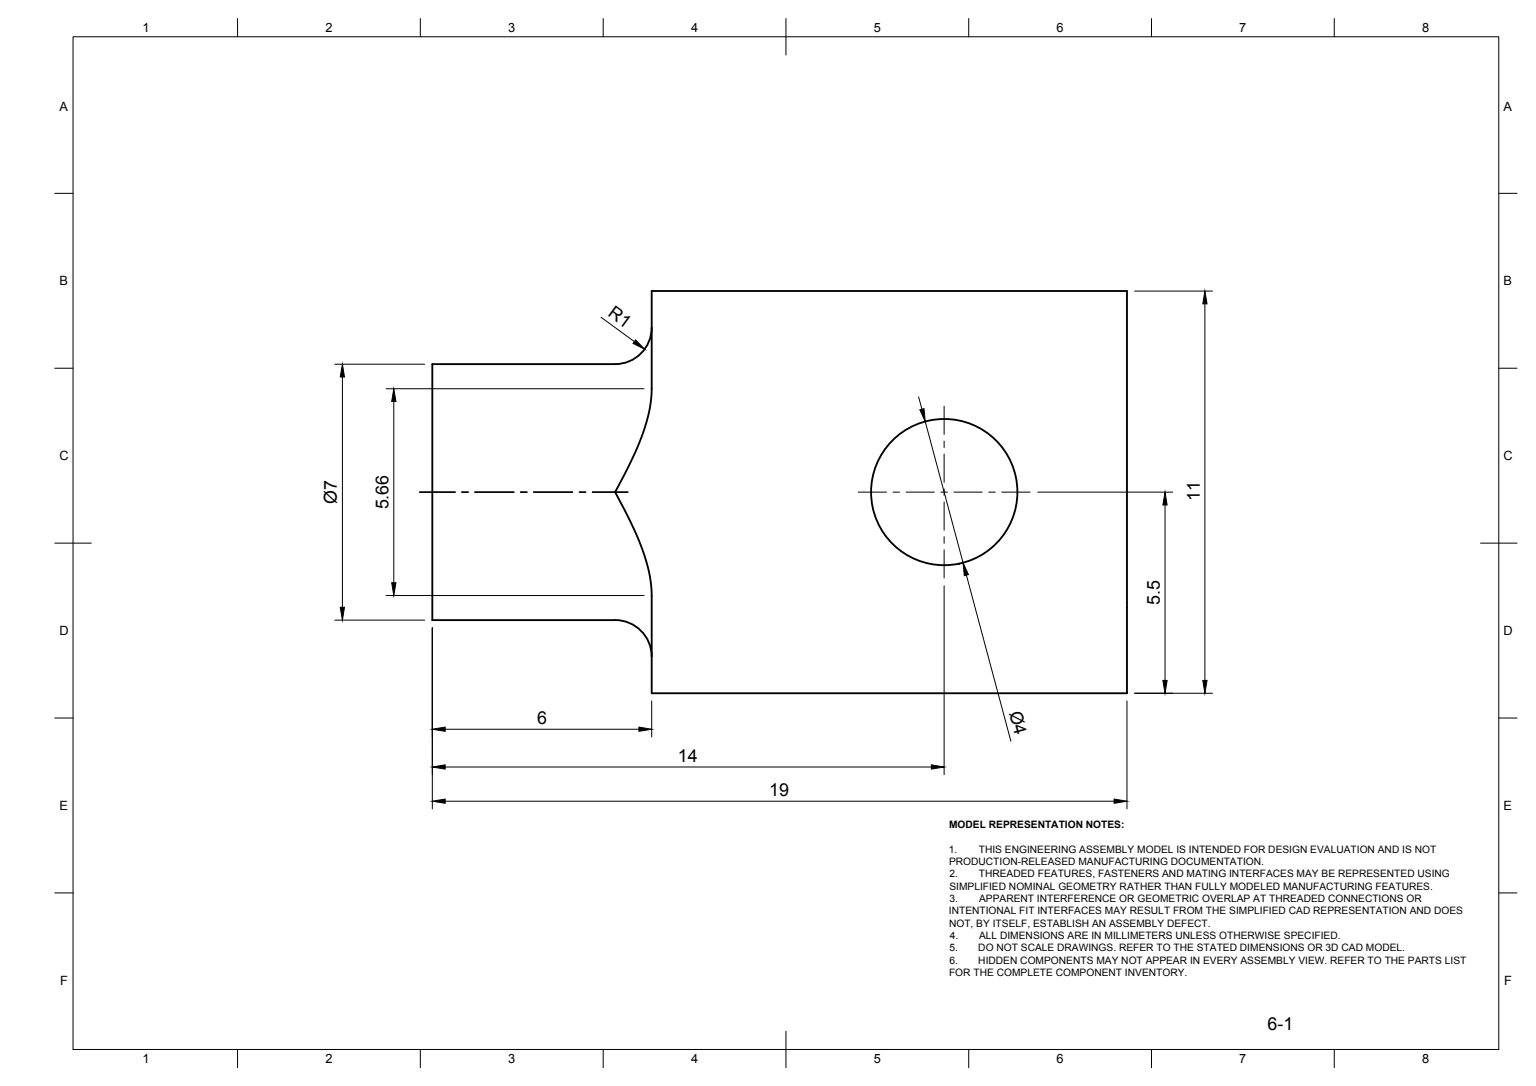
ISO-10303-21;
HEADER;
/* Generated by software containing ST-Developer
 * from STEP Tools, Inc. (www.steptools.com) 
 */

FILE_DESCRIPTION(
/* description */ (''),
/* implementation_level */ '2;1');

FILE_NAME(
/* name */ '6-1.step',
/* time_stamp */ '2026-10-06T01:16:10-07:00',
/* author */ (''),
/* organization */ (''),
/* preprocessor_version */ 'ST-DEVELOPER v20.2',
/* originating_system */ 'Autodesk Translation Framework v15.15.0.0',
/* authorisation */ '');

FILE_SCHEMA (('AUTOMOTIVE_DESIGN { 1 0 10303 214 3 1 1 }'));
ENDSEC;

DATA;
#10=MECHANICAL_DESIGN_GEOMETRIC_PRESENTATION_REPRESENTATION('',(#322,#323),#17113);
#144=TOROIDAL_SURFACE('',#6864,4.5,1.);
#145=TOROIDAL_SURFACE('',#6870,4.5,1.);
#217=B_SPLINE_CURVE_WITH_KNOTS('',3,(#16826,#16827,#16828,#16829),
 .UNSPECIFIED.,.F.,.F.,(4,4),(-0.288701302460675,0.),.UNSPECIFIED.);
#218=B_SPLINE_CURVE_WITH_KNOTS('',3,(#16830,#16831,#16832,#16833),
 .UNSPECIFIED.,.F.,.F.,(4,4),(-0.939904999188834,-0.651203696728158),
 .UNSPECIFIED.);
#219=B_SPLINE_CURVE_WITH_KNOTS('',3,(#16836,#16837,#16838,#16839),
 .UNSPECIFIED.,.F.,.F.,(4,4),(0.651203696728158,0.939904999188834),
 .UNSPECIFIED.);
#220=B_SPLINE_CURVE_WITH_KNOTS('',3,(#16849,#16850,#16851,#16852),
 .UNSPECIFIED.,.F.,.F.,(4,4),(0.,0.288701302460675),.UNSPECIFIED.);
#235=OPEN_SHELL('',(#5974,#5975));
#253=SHELL_BASED_SURFACE_MODEL('Body2',(#235));
#276=SHAPE_REPRESENTATION_RELATIONSHIP('SRR','None',#17202,#292);
#292=ADVANCED_BREP_SHAPE_REPRESENTATION('',(#342),#17109);
#322=STYLED_ITEM('',(#17298),#342);
#323=STYLED_ITEM('',(#17298),#253);
#342=MANIFOLD_SOLID_BREP('Body1',#6028);
#475=CYLINDRICAL_SURFACE('',#6844,2.);
#476=CYLINDRICAL_SURFACE('',#6857,1.75);
#477=CYLINDRICAL_SURFACE('',#6861,3.5);
#478=CYLINDRICAL_SURFACE('',#6867,2.);
#479=CYLINDRICAL_SURFACE('',#6871,2.);
#480=CYLINDRICAL_SURFACE('',#6872,5.5);
#481=CYLINDRICAL_SURFACE('',#6873,2.);
#482=CYLINDRICAL_SURFACE('',#6874,2.);
#483=CYLINDRICAL_SURFACE('',#6875,5.5);
#484=CYLINDRICAL_SURFACE('',#6876,2.);
#619=FACE_BOUND('',#1790,.T.);
#620=FACE_BOUND('',#1794,.T.);
#621=FACE_BOUND('',#1797,.T.);
#622=FACE_BOUND('',#1806,.T.);
#943=CIRCLE('',#6838,2.);
#944=CIRCLE('',#6839,5.5);
#945=CIRCLE('',#6840,2.);
#946=CIRCLE('',#6841,2.);
#947=CIRCLE('',#6842,5.5);
#948=CIRCLE('',#6843,2.);
#949=CIRCLE('',#6845,2.);
#950=CIRCLE('',#6847,1.75);
#951=CIRCLE('',#6849,4.5);
#952=CIRCLE('',#6850,2.);
#953=CIRCLE('',#6851,5.5);
#954=CIRCLE('',#6853,2.);
#955=CIRCLE('',#6854,4.5);
#956=CIRCLE('',#6855,2.);
#957=CIRCLE('',#6856,5.5);
#958=CIRCLE('',#6858,1.75);
#959=CIRCLE('',#6860,3.5);
#960=CIRCLE('',#6862,3.5);
#961=CIRCLE('',#6863,3.5);
#962=CIRCLE('',#6866,2.);
#963=CIRCLE('',#6868,2.);
#964=CIRCLE('',#6877,2.);
#965=CIRCLE('',#6878,2.);
#966=CIRCLE('',#6880,1.75);
#1308=FACE_OUTER_BOUND('',#1783,.T.);
#1309=FACE_OUTER_BOUND('',#1784,.T.);
#1310=FACE_OUTER_BOUND('',#1785,.T.);
#1311=FACE_OUTER_BOUND('',#1786,.T.);
#1312=FACE_OUTER_BOUND('',#1787,.T.);
#1313=FACE_OUTER_BOUND('',#1788,.T.);
#1314=FACE_OUTER_BOUND('',#1789,.T.);
#1315=FACE_OUTER_BOUND('',#1791,.T.);
#1316=FACE_OUTER_BOUND('',#1792,.T.);
#1317=FACE_OUTER_BOUND('',#1793,.T.);
#1318=FACE_OUTER_BOUND('',#1795,.T.);
#1319=FACE_OUTER_BOUND('',#1796,.T.);
#1320=FACE_OUTER_BOUND('',#1798,.T.);
#1321=FACE_OUTER_BOUND('',#1799,.T.);
#1322=FACE_OUTER_BOUND('',#1800,.T.);
#1323=FACE_OUTER_BOUND('',#1801,.T.);
#1324=FACE_OUTER_BOUND('',#1802,.T.);
#1325=FACE_OUTER_BOUND('',#1803,.T.);
#1326=FACE_OUTER_BOUND('',#1804,.T.);
#1327=FACE_OUTER_BOUND('',#1805,.T.);
#1783=EDGE_LOOP('',(#5252,#5253,#5254,#5255,#5256,#5257,#5258,#5259));
#1784=EDGE_LOOP('',(#5260,#5261,#5262,#5263));
#1785=EDGE_LOOP('',(#5264));
#1786=EDGE_LOOP('',(#5265,#5266,#5267,#5268,#5269,#5270));
#1787=EDGE_LOOP('',(#5271,#5272,#5273,#5274,#5275,#5276));
#1788=EDGE_LOOP('',(#5277,#5278,#5279,#5280));
#1789=EDGE_LOOP('',(#5281));
#1790=EDGE_LOOP('',(#5282));
#1791=EDGE_LOOP('',(#5283,#5284,#5285,#5286,#5287));
#1792=EDGE_LOOP('',(#5288,#5289,#5290,#5291));
#1793=EDGE_LOOP('',(#5292,#5293,#5294,#5295,#5296,#5297,#5298));
#1794=EDGE_LOOP('',(#5299));
#1795=EDGE_LOOP('',(#5300,#5301,#5302,#5303));
#1796=EDGE_LOOP('',(#5304,#5305,#5306,#5307,#5308,#5309,#5310));
#1797=EDGE_LOOP('',(#5311));
#1798=EDGE_LOOP('',(#5312,#5313,#5314,#5315));
#1799=EDGE_LOOP('',(#5316,#5317,#5318,#5319));
#1800=EDGE_LOOP('',(#5320,#5321,#5322,#5323));
#1801=EDGE_LOOP('',(#5324,#5325,#5326,#5327));
#1802=EDGE_LOOP('',(#5328,#5329,#5330,#5331));
#1803=EDGE_LOOP('',(#5332,#5333,#5334,#5335));
#1804=EDGE_LOOP('',(#5336,#5337,#5338,#5339));
#1805=EDGE_LOOP('',(#5340));
#1806=EDGE_LOOP('',(#5341));
#2160=LINE('',#16772,#2521);
#2161=LINE('',#16779,#2522);
#2162=LINE('',#16784,#2523);
#2163=LINE('',#16785,#2524);
#2164=LINE('',#16791,#2525);
#2165=LINE('',#16795,#2526);
#2166=LINE('',#16804,#2527);
#2167=LINE('',#16808,#2528);
#2168=LINE('',#16814,#2529);
#2169=LINE('',#16821,#2530);
#2170=LINE('',#16835,#2531);
#2171=LINE('',#16840,#2532);
#2172=LINE('',#16845,#2533);
#2173=LINE('',#16848,#2534);
#2174=LINE('',#16855,#2535);
#2175=LINE('',#16857,#2536);
#2176=LINE('',#16860,#2537);
#2177=LINE('',#16866,#2538);
#2521=VECTOR('',#8542,6.324555320337);
#2522=VECTOR('',#8549,6.324555320337);
#2523=VECTOR('',#8554,13.);
#2524=VECTOR('',#8555,13.);
#2525=VECTOR('',#8562,10.);
#2526=VECTOR('',#8565,10.);
#2527=VECTOR('',#8574,10.);
#2528=VECTOR('',#8577,10.);
#2529=VECTOR('',#8584,1.75);
#2530=VECTOR('',#8593,3.5);
#2531=VECTOR('',#8602,13.);
#2532=VECTOR('',#8603,13.);
#2533=VECTOR('',#8608,2.);
#2534=VECTOR('',#8613,13.);
#2535=VECTOR('',#8618,13.);
#2536=VECTOR('',#8621,13.);
#2537=VECTOR('',#8626,13.);
#2538=VECTOR('',#8633,2.);
#3017=VERTEX_POINT('',#16764);
#3018=VERTEX_POINT('',#16765);
#3019=VERTEX_POINT('',#16767);
#3020=VERTEX_POINT('',#16769);
#3021=VERTEX_POINT('',#16771);
#3022=VERTEX_POINT('',#16773);
#3023=VERTEX_POINT('',#16775);
#3024=VERTEX_POINT('',#16777);
#3025=VERTEX_POINT('',#16781);
#3026=VERTEX_POINT('',#16782);
#3027=VERTEX_POINT('',#16787);
#3028=VERTEX_POINT('',#16790);
#3029=VERTEX_POINT('',#16792);
#3030=VERTEX_POINT('',#16794);
#3031=VERTEX_POINT('',#16796);
#3032=VERTEX_POINT('',#16800);
#3033=VERTEX_POINT('',#16801);
#3034=VERTEX_POINT('',#16803);
#3035=VERTEX_POINT('',#16805);
#3036=VERTEX_POINT('',#16807);
#3037=VERTEX_POINT('',#16809);
#3038=VERTEX_POINT('',#16813);
#3039=VERTEX_POINT('',#16817);
#3040=VERTEX_POINT('',#16820);
#3041=VERTEX_POINT('',#16822);
#3042=VERTEX_POINT('',#16841);
#3043=VERTEX_POINT('',#16844);
#3044=VERTEX_POINT('',#16863);
#3045=VERTEX_POINT('',#16865);
#3046=VERTEX_POINT('',#16869);
#3786=EDGE_CURVE('',#3017,#3018,#943,.T.);
#3787=EDGE_CURVE('',#3018,#3019,#944,.T.);
#3788=EDGE_CURVE('',#3019,#3020,#945,.T.);
#3789=EDGE_CURVE('',#3020,#3021,#2160,.T.);
#3790=EDGE_CURVE('',#3021,#3022,#946,.T.);
#3791=EDGE_CURVE('',#3022,#3023,#947,.T.);
#3792=EDGE_CURVE('',#3023,#3024,#948,.T.);
#3793=EDGE_CURVE('',#3024,#3017,#2161,.T.);
#3794=EDGE_CURVE('',#3025,#3026,#949,.T.);
#3795=EDGE_CURVE('',#3018,#3025,#2162,.T.);
#3796=EDGE_CURVE('',#3017,#3026,#2163,.T.);
#3797=EDGE_CURVE('',#3027,#3027,#950,.T.);
#3798=EDGE_CURVE('',#3028,#3026,#2164,.T.);
#3799=EDGE_CURVE('',#3029,#3028,#951,.T.);
#3800=EDGE_CURVE('',#3030,#3029,#2165,.T.);
#3801=EDGE_CURVE('',#3030,#3031,#952,.T.);
#3802=EDGE_CURVE('',#3025,#3031,#953,.T.);
#3803=EDGE_CURVE('',#3032,#3033,#954,.T.);
#3804=EDGE_CURVE('',#3034,#3033,#2166,.T.);
#3805=EDGE_CURVE('',#3035,#3034,#955,.T.);
#3806=EDGE_CURVE('',#3036,#3035,#2167,.T.);
#3807=EDGE_CURVE('',#3036,#3037,#956,.T.);
#3808=EDGE_CURVE('',#3032,#3037,#957,.T.);
#3809=EDGE_CURVE('',#3027,#3038,#2168,.T.);
#3810=EDGE_CURVE('',#3038,#3038,#958,.T.);
#3811=EDGE_CURVE('',#3039,#3039,#959,.T.);
#3812=EDGE_CURVE('',#3039,#3040,#2169,.T.);
#3813=EDGE_CURVE('',#3040,#3041,#960,.T.);
#3814=EDGE_CURVE('',#3041,#3040,#961,.T.);
#3815=EDGE_CURVE('',#3028,#3040,#217,.T.);
#3816=EDGE_CURVE('',#3041,#3029,#218,.T.);
#3817=EDGE_CURVE('',#3020,#3030,#2170,.T.);
#3818=EDGE_CURVE('',#3034,#3041,#219,.T.);
#3819=EDGE_CURVE('',#3021,#3033,#2171,.T.);
#3820=EDGE_CURVE('',#3042,#3042,#962,.T.);
#3821=EDGE_CURVE('',#3042,#3043,#2172,.T.);
#3822=EDGE_CURVE('',#3043,#3043,#963,.T.);
#3823=EDGE_CURVE('',#3024,#3036,#2173,.T.);
#3824=EDGE_CURVE('',#3040,#3035,#220,.T.);
#3825=EDGE_CURVE('',#3023,#3037,#2174,.T.);
#3826=EDGE_CURVE('',#3022,#3032,#2175,.T.);
#3827=EDGE_CURVE('',#3019,#3031,#2176,.T.);
#3828=EDGE_CURVE('',#3044,#3044,#964,.T.);
#3829=EDGE_CURVE('',#3044,#3045,#2177,.T.);
#3830=EDGE_CURVE('',#3045,#3045,#965,.T.);
#3831=EDGE_CURVE('',#3046,#3046,#966,.T.);
#5252=ORIENTED_EDGE('',*,*,#3786,.T.);
#5253=ORIENTED_EDGE('',*,*,#3787,.T.);
#5254=ORIENTED_EDGE('',*,*,#3788,.T.);
#5255=ORIENTED_EDGE('',*,*,#3789,.T.);
#5256=ORIENTED_EDGE('',*,*,#3790,.T.);
#5257=ORIENTED_EDGE('',*,*,#3791,.T.);
#5258=ORIENTED_EDGE('',*,*,#3792,.T.);
#5259=ORIENTED_EDGE('',*,*,#3793,.T.);
#5260=ORIENTED_EDGE('',*,*,#3794,.F.);
#5261=ORIENTED_EDGE('',*,*,#3795,.F.);
#5262=ORIENTED_EDGE('',*,*,#3786,.F.);
#5263=ORIENTED_EDGE('',*,*,#3796,.T.);
#5264=ORIENTED_EDGE('',*,*,#3797,.T.);
#5265=ORIENTED_EDGE('',*,*,#3794,.T.);
#5266=ORIENTED_EDGE('',*,*,#3798,.F.);
#5267=ORIENTED_EDGE('',*,*,#3799,.F.);
#5268=ORIENTED_EDGE('',*,*,#3800,.F.);
#5269=ORIENTED_EDGE('',*,*,#3801,.T.);
#5270=ORIENTED_EDGE('',*,*,#3802,.F.);
#5271=ORIENTED_EDGE('',*,*,#3803,.T.);
#5272=ORIENTED_EDGE('',*,*,#3804,.F.);
#5273=ORIENTED_EDGE('',*,*,#3805,.F.);
#5274=ORIENTED_EDGE('',*,*,#3806,.F.);
#5275=ORIENTED_EDGE('',*,*,#3807,.T.);
#5276=ORIENTED_EDGE('',*,*,#3808,.F.);
#5277=ORIENTED_EDGE('',*,*,#3797,.F.);
#5278=ORIENTED_EDGE('',*,*,#3809,.T.);
#5279=ORIENTED_EDGE('',*,*,#3810,.F.);
#5280=ORIENTED_EDGE('',*,*,#3809,.F.);
#5281=ORIENTED_EDGE('',*,*,#3811,.T.);
#5282=ORIENTED_EDGE('',*,*,#3810,.T.);
#5283=ORIENTED_EDGE('',*,*,#3811,.F.);
#5284=ORIENTED_EDGE('',*,*,#3812,.T.);
#5285=ORIENTED_EDGE('',*,*,#3813,.T.);
#5286=ORIENTED_EDGE('',*,*,#3814,.T.);
#5287=ORIENTED_EDGE('',*,*,#3812,.F.);
#5288=ORIENTED_EDGE('',*,*,#3799,.T.);
#5289=ORIENTED_EDGE('',*,*,#3815,.T.);
#5290=ORIENTED_EDGE('',*,*,#3814,.F.);
#5291=ORIENTED_EDGE('',*,*,#3816,.T.);
#5292=ORIENTED_EDGE('',*,*,#3817,.T.);
#5293=ORIENTED_EDGE('',*,*,#3800,.T.);
#5294=ORIENTED_EDGE('',*,*,#3816,.F.);
#5295=ORIENTED_EDGE('',*,*,#3818,.F.);
#5296=ORIENTED_EDGE('',*,*,#3804,.T.);
#5297=ORIENTED_EDGE('',*,*,#3819,.F.);
#5298=ORIENTED_EDGE('',*,*,#3789,.F.);
#5299=ORIENTED_EDGE('',*,*,#3820,.T.);
#5300=ORIENTED_EDGE('',*,*,#3820,.F.);
#5301=ORIENTED_EDGE('',*,*,#3821,.T.);
#5302=ORIENTED_EDGE('',*,*,#3822,.T.);
#5303=ORIENTED_EDGE('',*,*,#3821,.F.);
#5304=ORIENTED_EDGE('',*,*,#3796,.F.);
#5305=ORIENTED_EDGE('',*,*,#3793,.F.);
#5306=ORIENTED_EDGE('',*,*,#3823,.T.);
#5307=ORIENTED_EDGE('',*,*,#3806,.T.);
#5308=ORIENTED_EDGE('',*,*,#3824,.F.);
#5309=ORIENTED_EDGE('',*,*,#3815,.F.);
#5310=ORIENTED_EDGE('',*,*,#3798,.T.);
#5311=ORIENTED_EDGE('',*,*,#3822,.F.);
#5312=ORIENTED_EDGE('',*,*,#3813,.F.);
#5313=ORIENTED_EDGE('',*,*,#3824,.T.);
#5314=ORIENTED_EDGE('',*,*,#3805,.T.);
#5315=ORIENTED_EDGE('',*,*,#3818,.T.);
#5316=ORIENTED_EDGE('',*,*,#3807,.F.);
#5317=ORIENTED_EDGE('',*,*,#3823,.F.);
#5318=ORIENTED_EDGE('',*,*,#3792,.F.);
#5319=ORIENTED_EDGE('',*,*,#3825,.T.);
#5320=ORIENTED_EDGE('',*,*,#3826,.T.);
#5321=ORIENTED_EDGE('',*,*,#3808,.T.);
#5322=ORIENTED_EDGE('',*,*,#3825,.F.);
#5323=ORIENTED_EDGE('',*,*,#3791,.F.);
#5324=ORIENTED_EDGE('',*,*,#3803,.F.);
#5325=ORIENTED_EDGE('',*,*,#3826,.F.);
#5326=ORIENTED_EDGE('',*,*,#3790,.F.);
#5327=ORIENTED_EDGE('',*,*,#3819,.T.);
#5328=ORIENTED_EDGE('',*,*,#3801,.F.);
#5329=ORIENTED_EDGE('',*,*,#3817,.F.);
#5330=ORIENTED_EDGE('',*,*,#3788,.F.);
#5331=ORIENTED_EDGE('',*,*,#3827,.T.);
#5332=ORIENTED_EDGE('',*,*,#3795,.T.);
#5333=ORIENTED_EDGE('',*,*,#3802,.T.);
#5334=ORIENTED_EDGE('',*,*,#3827,.F.);
#5335=ORIENTED_EDGE('',*,*,#3787,.F.);
#5336=ORIENTED_EDGE('',*,*,#3828,.F.);
#5337=ORIENTED_EDGE('',*,*,#3829,.T.);
#5338=ORIENTED_EDGE('',*,*,#3830,.T.);
#5339=ORIENTED_EDGE('',*,*,#3829,.F.);
#5340=ORIENTED_EDGE('',*,*,#3830,.F.);
#5341=ORIENTED_EDGE('',*,*,#3831,.F.);
#5627=PLANE('',#6837);
#5628=PLANE('',#6846);
#5629=PLANE('',#6848);
#5630=PLANE('',#6852);
#5631=PLANE('',#6859);
#5632=PLANE('',#6865);
#5633=PLANE('',#6869);
#5634=PLANE('',#6879);
#5956=ADVANCED_FACE('',(#1308),#5627,.T.);
#5957=ADVANCED_FACE('',(#1309),#475,.T.);
#5958=ADVANCED_FACE('',(#1310),#5628,.F.);
#5959=ADVANCED_FACE('',(#1311),#5629,.F.);
#5960=ADVANCED_FACE('',(#1312),#5630,.F.);
#5961=ADVANCED_FACE('',(#1313),#476,.F.);
#5962=ADVANCED_FACE('',(#1314,#619),#5631,.T.);
#5963=ADVANCED_FACE('',(#1315),#477,.T.);
#5964=ADVANCED_FACE('',(#1316),#144,.F.);
#5965=ADVANCED_FACE('',(#1317,#620),#5632,.T.);
#5966=ADVANCED_FACE('',(#1318),#478,.F.);
#5967=ADVANCED_FACE('',(#1319,#621),#5633,.T.);
#5968=ADVANCED_FACE('',(#1320),#145,.F.);
#5969=ADVANCED_FACE('',(#1321),#479,.T.);
#5970=ADVANCED_FACE('',(#1322),#480,.T.);
#5971=ADVANCED_FACE('',(#1323),#481,.T.);
#5972=ADVANCED_FACE('',(#1324),#482,.T.);
#5973=ADVANCED_FACE('',(#1325),#483,.T.);
#5974=ADVANCED_FACE('',(#1326),#484,.T.);
#5975=ADVANCED_FACE('',(#1327,#622),#5634,.F.);
#6028=CLOSED_SHELL('',(#5956,#5957,#5958,#5959,#5960,#5961,#5962,#5963,
#5964,#5965,#5966,#5967,#5968,#5969,#5970,#5971,#5972,#5973));
#6836=AXIS2_PLACEMENT_3D('',#16762,#8532,#8533);
#6837=AXIS2_PLACEMENT_3D('',#16763,#8534,#8535);
#6838=AXIS2_PLACEMENT_3D('',#16766,#8536,#8537);
#6839=AXIS2_PLACEMENT_3D('',#16768,#8538,#8539);
#6840=AXIS2_PLACEMENT_3D('',#16770,#8540,#8541);
#6841=AXIS2_PLACEMENT_3D('',#16774,#8543,#8544);
#6842=AXIS2_PLACEMENT_3D('',#16776,#8545,#8546);
#6843=AXIS2_PLACEMENT_3D('',#16778,#8547,#8548);
#6844=AXIS2_PLACEMENT_3D('',#16780,#8550,#8551);
#6845=AXIS2_PLACEMENT_3D('',#16783,#8552,#8553);
#6846=AXIS2_PLACEMENT_3D('',#16786,#8556,#8557);
#6847=AXIS2_PLACEMENT_3D('',#16788,#8558,#8559);
#6848=AXIS2_PLACEMENT_3D('',#16789,#8560,#8561);
#6849=AXIS2_PLACEMENT_3D('',#16793,#8563,#8564);
#6850=AXIS2_PLACEMENT_3D('',#16797,#8566,#8567);
#6851=AXIS2_PLACEMENT_3D('',#16798,#8568,#8569);
#6852=AXIS2_PLACEMENT_3D('',#16799,#8570,#8571);
#6853=AXIS2_PLACEMENT_3D('',#16802,#8572,#8573);
#6854=AXIS2_PLACEMENT_3D('',#16806,#8575,#8576);
#6855=AXIS2_PLACEMENT_3D('',#16810,#8578,#8579);
#6856=AXIS2_PLACEMENT_3D('',#16811,#8580,#8581);
#6857=AXIS2_PLACEMENT_3D('',#16812,#8582,#8583);
#6858=AXIS2_PLACEMENT_3D('',#16815,#8585,#8586);
#6859=AXIS2_PLACEMENT_3D('',#16816,#8587,#8588);
#6860=AXIS2_PLACEMENT_3D('',#16818,#8589,#8590);
#6861=AXIS2_PLACEMENT_3D('',#16819,#8591,#8592);
#6862=AXIS2_PLACEMENT_3D('',#16823,#8594,#8595);
#6863=AXIS2_PLACEMENT_3D('',#16824,#8596,#8597);
#6864=AXIS2_PLACEMENT_3D('',#16825,#8598,#8599);
#6865=AXIS2_PLACEMENT_3D('',#16834,#8600,#8601);
#6866=AXIS2_PLACEMENT_3D('',#16842,#8604,#8605);
#6867=AXIS2_PLACEMENT_3D('',#16843,#8606,#8607);
#6868=AXIS2_PLACEMENT_3D('',#16846,#8609,#8610);
#6869=AXIS2_PLACEMENT_3D('',#16847,#8611,#8612);
#6870=AXIS2_PLACEMENT_3D('',#16853,#8614,#8615);
#6871=AXIS2_PLACEMENT_3D('',#16854,#8616,#8617);
#6872=AXIS2_PLACEMENT_3D('',#16856,#8619,#8620);
#6873=AXIS2_PLACEMENT_3D('',#16858,#8622,#8623);
#6874=AXIS2_PLACEMENT_3D('',#16859,#8624,#8625);
#6875=AXIS2_PLACEMENT_3D('',#16861,#8627,#8628);
#6876=AXIS2_PLACEMENT_3D('',#16862,#8629,#8630);
#6877=AXIS2_PLACEMENT_3D('',#16864,#8631,#8632);
#6878=AXIS2_PLACEMENT_3D('',#16867,#8634,#8635);
#6879=AXIS2_PLACEMENT_3D('',#16868,#8636,#8637);
#6880=AXIS2_PLACEMENT_3D('',#16870,#8638,#8639);
#8532=DIRECTION('axis',(0.,0.,1.));
#8533=DIRECTION('refdir',(1.,0.,0.));
#8534=DIRECTION('center_axis',(0.,1.,0.));
#8535=DIRECTION('ref_axis',(1.,0.,0.));
#8536=DIRECTION('center_axis',(0.,1.,0.));
#8537=DIRECTION('ref_axis',(0.,0.,1.));
#8538=DIRECTION('center_axis',(0.,1.,0.));
#8539=DIRECTION('ref_axis',(0.903507902905271,0.,0.428571428571386));
#8540=DIRECTION('center_axis',(0.,1.,0.));
#8541=DIRECTION('ref_axis',(0.903507902905271,0.,-0.428571428571386));
#8542=DIRECTION('',(-1.,0.,0.));
#8543=DIRECTION('center_axis',(0.,1.,0.));
#8544=DIRECTION('ref_axis',(0.,0.,-1.));
#8545=DIRECTION('center_axis',(0.,1.,0.));
#8546=DIRECTION('ref_axis',(-0.903507902905271,0.,-0.428571428571386));
#8547=DIRECTION('center_axis',(0.,1.,0.));
#8548=DIRECTION('ref_axis',(-0.903507902905271,0.,0.428571428571386));
#8549=DIRECTION('',(1.,0.,0.));
#8550=DIRECTION('center_axis',(0.,-1.,0.));
#8551=DIRECTION('ref_axis',(0.903507902905271,0.,0.428571428571386));
#8552=DIRECTION('center_axis',(0.,-1.,0.));
#8553=DIRECTION('ref_axis',(0.903507902905271,0.,0.428571428571386));
#8554=DIRECTION('',(0.,-1.,0.));
#8555=DIRECTION('',(0.,-1.,0.));
#8556=DIRECTION('center_axis',(0.,1.,0.));
#8557=DIRECTION('ref_axis',(1.,0.,0.));
#8558=DIRECTION('center_axis',(0.,-1.,0.));
#8559=DIRECTION('ref_axis',(0.,0.,1.));
#8560=DIRECTION('center_axis',(0.,1.,0.));
#8561=DIRECTION('ref_axis',(1.,0.,0.));
#8562=DIRECTION('',(1.,0.,0.));
#8563=DIRECTION('center_axis',(0.,-1.,0.));
#8564=DIRECTION('ref_axis',(0.628539361054693,0.,-0.777777777777791));
#8565=DIRECTION('',(-1.,0.,0.));
#8566=DIRECTION('center_axis',(0.,-1.,0.));
#8567=DIRECTION('ref_axis',(0.,0.,-1.));
#8568=DIRECTION('center_axis',(0.,1.,0.));
#8569=DIRECTION('ref_axis',(0.903507902905271,0.,0.428571428571386));
#8570=DIRECTION('center_axis',(0.,1.,0.));
#8571=DIRECTION('ref_axis',(1.,0.,0.));
#8572=DIRECTION('center_axis',(0.,-1.,0.));
#8573=DIRECTION('ref_axis',(-0.903507902905271,0.,-0.428571428571386));
#8574=DIRECTION('',(-1.,0.,0.));
#8575=DIRECTION('center_axis',(0.,-1.,0.));
#8576=DIRECTION('ref_axis',(-0.628539361054693,0.,0.777777777777791));
#8577=DIRECTION('',(1.,0.,0.));
#8578=DIRECTION('center_axis',(0.,-1.,0.));
#8579=DIRECTION('ref_axis',(0.,0.,1.));
#8580=DIRECTION('center_axis',(0.,1.,0.));
#8581=DIRECTION('ref_axis',(-0.903507902905271,0.,-0.428571428571386));
#8582=DIRECTION('center_axis',(0.,-1.,0.));
#8583=DIRECTION('ref_axis',(0.,0.,-1.));
#8584=DIRECTION('',(0.,-1.,0.));
#8585=DIRECTION('center_axis',(0.,1.,0.));
#8586=DIRECTION('ref_axis',(0.,0.,-1.));
#8587=DIRECTION('center_axis',(0.,-1.,0.));
#8588=DIRECTION('ref_axis',(0.,0.,-1.));
#8589=DIRECTION('center_axis',(0.,-1.,0.));
#8590=DIRECTION('ref_axis',(0.,0.,-1.));
#8591=DIRECTION('center_axis',(0.,-1.,0.));
#8592=DIRECTION('ref_axis',(0.,0.,-1.));
#8593=DIRECTION('',(0.,1.,0.));
#8594=DIRECTION('center_axis',(0.,-1.,0.));
#8595=DIRECTION('ref_axis',(0.,0.,1.));
#8596=DIRECTION('center_axis',(0.,-1.,0.));
#8597=DIRECTION('ref_axis',(0.,0.,-1.));
#8598=DIRECTION('center_axis',(0.,-1.,0.));
#8599=DIRECTION('ref_axis',(1.,0.,-1.75640751942652E-17));
#8600=DIRECTION('center_axis',(0.,0.,-1.));
#8601=DIRECTION('ref_axis',(-1.,0.,0.));
#8602=DIRECTION('',(0.,-1.,0.));
#8603=DIRECTION('',(0.,-1.,0.));
#8604=DIRECTION('center_axis',(0.,0.,1.));
#8605=DIRECTION('ref_axis',(0.,-1.,0.));
#8606=DIRECTION('center_axis',(0.,0.,1.));
#8607=DIRECTION('ref_axis',(0.,-1.,0.));
#8608=DIRECTION('',(0.,0.,1.));
#8609=DIRECTION('center_axis',(0.,0.,1.));
#8610=DIRECTION('ref_axis',(0.,-1.,0.));
#8611=DIRECTION('center_axis',(0.,0.,1.));
#8612=DIRECTION('ref_axis',(1.,0.,0.));
#8613=DIRECTION('',(0.,-1.,0.));
#8614=DIRECTION('center_axis',(0.,-1.,0.));
#8615=DIRECTION('ref_axis',(-1.,0.,-2.27465615787459E-16));
#8616=DIRECTION('center_axis',(0.,-1.,0.));
#8617=DIRECTION('ref_axis',(0.,0.,1.));
#8618=DIRECTION('',(0.,-1.,0.));
#8619=DIRECTION('center_axis',(0.,1.,0.));
#8620=DIRECTION('ref_axis',(-1.,0.,-1.22464679914735E-16));
#8621=DIRECTION('',(0.,-1.,0.));
#8622=DIRECTION('center_axis',(0.,-1.,0.));
#8623=DIRECTION('ref_axis',(-0.903507902905271,0.,-0.428571428571386));
#8624=DIRECTION('center_axis',(0.,-1.,0.));
#8625=DIRECTION('ref_axis',(0.,0.,-1.));
#8626=DIRECTION('',(0.,-1.,0.));
#8627=DIRECTION('center_axis',(0.,1.,0.));
#8628=DIRECTION('ref_axis',(1.,0.,0.));
#8629=DIRECTION('center_axis',(0.,-1.,0.));
#8630=DIRECTION('ref_axis',(1.,0.,0.));
#8631=DIRECTION('center_axis',(0.,-1.,0.));
#8632=DIRECTION('ref_axis',(-1.,0.,0.));
#8633=DIRECTION('',(0.,1.,0.));
#8634=DIRECTION('center_axis',(0.,-1.,0.));
#8635=DIRECTION('ref_axis',(-1.,0.,0.));
#8636=DIRECTION('center_axis',(0.,-1.,0.));
#8637=DIRECTION('ref_axis',(1.,0.,0.));
#8638=DIRECTION('center_axis',(0.,1.,0.));
#8639=DIRECTION('ref_axis',(-1.,0.,0.));
#16762=CARTESIAN_POINT('',(0.,0.,0.));
#16763=CARTESIAN_POINT('Origin',(0.,0.,0.));
#16764=CARTESIAN_POINT('',(3.162277660168,0.,3.5));
#16765=CARTESIAN_POINT('',(4.969293465979,0.,2.357142857143));
#16766=CARTESIAN_POINT('Origin',(3.162277660168,0.,1.5));
#16767=CARTESIAN_POINT('',(4.969293465979,0.,-2.357142857143));
#16768=CARTESIAN_POINT('Origin',(0.,0.,0.));
#16769=CARTESIAN_POINT('',(3.162277660168,0.,-3.5));
#16770=CARTESIAN_POINT('Origin',(3.162277660168,0.,-1.5));
#16771=CARTESIAN_POINT('',(-3.162277660168,0.,-3.5));
#16772=CARTESIAN_POINT('',(3.162277660168,0.,-3.5));
#16773=CARTESIAN_POINT('',(-4.969293465979,0.,-2.357142857143));
#16774=CARTESIAN_POINT('Origin',(-3.162277660168,0.,-1.5));
#16775=CARTESIAN_POINT('',(-4.969293465979,0.,2.357142857143));
#16776=CARTESIAN_POINT('Origin',(0.,0.,0.));
#16777=CARTESIAN_POINT('',(-3.162277660168,0.,3.5));
#16778=CARTESIAN_POINT('Origin',(-3.162277660168,0.,1.5));
#16779=CARTESIAN_POINT('',(-3.162277660168,0.,3.5));
#16780=CARTESIAN_POINT('Origin',(3.162277660168,24.7684,1.5));
#16781=CARTESIAN_POINT('',(4.969293465979,-13.,2.357142857143));
#16782=CARTESIAN_POINT('',(3.162277660168,-13.,3.5));
#16783=CARTESIAN_POINT('Origin',(3.162277660168,-13.,1.5));
#16784=CARTESIAN_POINT('',(4.969293465979,0.,2.357142857143));
#16785=CARTESIAN_POINT('',(3.162277660168,0.,3.5));
#16786=CARTESIAN_POINT('Origin',(0.,-13.,0.));
#16787=CARTESIAN_POINT('',(-2.14313189850787E-16,-13.,1.75));
#16788=CARTESIAN_POINT('Origin',(0.,-13.,0.));
#16789=CARTESIAN_POINT('Origin',(0.,-13.,0.));
#16790=CARTESIAN_POINT('',(2.828427124746,-13.,3.5));
#16791=CARTESIAN_POINT('',(-2.1213203435595,-13.,3.5));
#16792=CARTESIAN_POINT('',(2.828427124746,-13.,-3.5));
#16793=CARTESIAN_POINT('Origin',(0.,-13.,0.));
#16794=CARTESIAN_POINT('',(3.162277660168,-13.,-3.5));
#16795=CARTESIAN_POINT('',(2.1213203435595,-13.,-3.5));
#16796=CARTESIAN_POINT('',(4.969293465979,-13.,-2.357142857143));
#16797=CARTESIAN_POINT('Origin',(3.162277660168,-13.,-1.5));
#16798=CARTESIAN_POINT('Origin',(0.,-13.,0.));
#16799=CARTESIAN_POINT('Origin',(0.,-13.,0.));
#16800=CARTESIAN_POINT('',(-4.969293465979,-13.,-2.357142857143));
#16801=CARTESIAN_POINT('',(-3.162277660168,-13.,-3.5));
#16802=CARTESIAN_POINT('Origin',(-3.162277660168,-13.,-1.5));
#16803=CARTESIAN_POINT('',(-2.828427124746,-13.,-3.5));
#16804=CARTESIAN_POINT('',(2.1213203435595,-13.,-3.5));
#16805=CARTESIAN_POINT('',(-2.828427124746,-13.,3.5));
#16806=CARTESIAN_POINT('Origin',(0.,-13.,0.));
#16807=CARTESIAN_POINT('',(-3.162277660168,-13.,3.5));
#16808=CARTESIAN_POINT('',(-2.1213203435595,-13.,3.5));
#16809=CARTESIAN_POINT('',(-4.969293465979,-13.,2.357142857143));
#16810=CARTESIAN_POINT('Origin',(-3.162277660168,-13.,1.5));
#16811=CARTESIAN_POINT('Origin',(0.,-13.,0.));
#16812=CARTESIAN_POINT('Origin',(0.,-13.,0.));
#16813=CARTESIAN_POINT('',(-2.14313189850787E-16,-19.,1.75));
#16814=CARTESIAN_POINT('',(-2.14313189850787E-16,-13.,1.75));
#16815=CARTESIAN_POINT('Origin',(0.,-19.,0.));
#16816=CARTESIAN_POINT('Origin',(0.,-19.,0.));
#16817=CARTESIAN_POINT('',(-4.28626379701574E-16,-19.,3.5));
#16818=CARTESIAN_POINT('Origin',(0.,-19.,0.));
#16819=CARTESIAN_POINT('Origin',(0.,-13.,0.));
#16820=CARTESIAN_POINT('',(0.,-14.,3.5));
#16821=CARTESIAN_POINT('',(-4.28626379701574E-16,-13.,3.5));
#16822=CARTESIAN_POINT('',(0.,-14.,-3.5));
#16823=CARTESIAN_POINT('Origin',(0.,-14.,0.));
#16824=CARTESIAN_POINT('Origin',(0.,-14.,0.));
#16825=CARTESIAN_POINT('Origin',(0.,-14.,0.));
#16826=CARTESIAN_POINT('Ctrl Pts',(2.82842712474619,-13.,3.5));
#16827=CARTESIAN_POINT('Ctrl Pts',(1.86608944987721,-13.0000000000001,3.5));
#16828=CARTESIAN_POINT('Ctrl Pts',(0.848702054990486,-13.5463496695392,
3.5));
#16829=CARTESIAN_POINT('Ctrl Pts',(0.,-14.,3.5));
#16830=CARTESIAN_POINT('Ctrl Pts',(0.,-14.,-3.5));
#16831=CARTESIAN_POINT('Ctrl Pts',(0.848702054990486,-13.5463496695392,
-3.5));
#16832=CARTESIAN_POINT('Ctrl Pts',(1.86608944987721,-13.,-3.5));
#16833=CARTESIAN_POINT('Ctrl Pts',(2.82842712474619,-13.,-3.5));
#16834=CARTESIAN_POINT('Origin',(4.242640687119,0.,-3.5));
#16835=CARTESIAN_POINT('',(3.162277660168,0.,-3.5));
#16836=CARTESIAN_POINT('Ctrl Pts',(-2.82842712474619,-13.,-3.5));
#16837=CARTESIAN_POINT('Ctrl Pts',(-1.86608944987721,-13.0000000000001,
-3.5));
#16838=CARTESIAN_POINT('Ctrl Pts',(-0.848702054990486,-13.5463496695392,
-3.5));
#16839=CARTESIAN_POINT('Ctrl Pts',(0.,-14.,-3.5));
#16840=CARTESIAN_POINT('',(-3.162277660168,0.,-3.5));
#16841=CARTESIAN_POINT('',(-2.44929359829471E-16,-3.,-3.5));
#16842=CARTESIAN_POINT('Origin',(0.,-5.,-3.5));
#16843=CARTESIAN_POINT('Origin',(0.,-5.,-4.8));
#16844=CARTESIAN_POINT('',(-2.44929359829471E-16,-3.,3.5));
#16845=CARTESIAN_POINT('',(-2.44929359829471E-16,-3.,-4.8));
#16846=CARTESIAN_POINT('Origin',(0.,-5.,3.5));
#16847=CARTESIAN_POINT('Origin',(-4.242640687119,0.,3.5));
#16848=CARTESIAN_POINT('',(-3.162277660168,0.,3.5));
#16849=CARTESIAN_POINT('Ctrl Pts',(0.,-14.,3.5));
#16850=CARTESIAN_POINT('Ctrl Pts',(-0.848702054990486,-13.5463496695392,
3.5));
#16851=CARTESIAN_POINT('Ctrl Pts',(-1.86608944987721,-13.,3.5));
#16852=CARTESIAN_POINT('Ctrl Pts',(-2.82842712474619,-13.,3.5));
#16853=CARTESIAN_POINT('Origin',(0.,-14.,0.));
#16854=CARTESIAN_POINT('Origin',(-3.162277660168,24.7684,1.5));
#16855=CARTESIAN_POINT('',(-4.969293465979,0.,2.357142857143));
#16856=CARTESIAN_POINT('Origin',(0.,0.,0.));
#16857=CARTESIAN_POINT('',(-4.969293465979,0.,-2.357142857143));
#16858=CARTESIAN_POINT('Origin',(-3.162277660168,24.7684,-1.5));
#16859=CARTESIAN_POINT('Origin',(3.162277660168,24.7684,-1.5));
#16860=CARTESIAN_POINT('',(4.969293465979,0.,-2.357142857143));
#16861=CARTESIAN_POINT('Origin',(0.,0.,0.));
#16862=CARTESIAN_POINT('Origin',(0.,-19.,0.));
#16863=CARTESIAN_POINT('',(-2.,-19.,-2.44929359829471E-16));
#16864=CARTESIAN_POINT('Origin',(0.,-19.,0.));
#16865=CARTESIAN_POINT('',(-2.,-13.,-2.44929359829471E-16));
#16866=CARTESIAN_POINT('',(-2.,-19.,-2.44929359829471E-16));
#16867=CARTESIAN_POINT('Origin',(0.,-13.,0.));
#16868=CARTESIAN_POINT('Origin',(0.,-13.,0.));
#16869=CARTESIAN_POINT('',(1.75,-13.,0.));
#16870=CARTESIAN_POINT('Origin',(0.,-13.,0.));
#17086=UNCERTAINTY_MEASURE_WITH_UNIT(LENGTH_MEASURE(0.01),#17114,
'DISTANCE_ACCURACY_VALUE',
'Maximum model space distance between geometric entities at asserted c
onnectivities');
#17090=UNCERTAINTY_MEASURE_WITH_UNIT(LENGTH_MEASURE(0.01),#17114,
'DISTANCE_ACCURACY_VALUE',
'Maximum model space distance between geometric entities at asserted c
onnectivities');
#17109=(
GEOMETRIC_REPRESENTATION_CONTEXT(3)
GLOBAL_UNCERTAINTY_ASSIGNED_CONTEXT((#17086))
GLOBAL_UNIT_ASSIGNED_CONTEXT((#17114,#17116,#17117))
REPRESENTATION_CONTEXT('','3D')
);
#17113=(
GEOMETRIC_REPRESENTATION_CONTEXT(3)
GLOBAL_UNCERTAINTY_ASSIGNED_CONTEXT((#17090))
GLOBAL_UNIT_ASSIGNED_CONTEXT((#17114,#17116,#17117))
REPRESENTATION_CONTEXT('','3D')
);
#17114=(
LENGTH_UNIT()
NAMED_UNIT(*)
SI_UNIT(.MILLI.,.METRE.)
);
#17116=(
NAMED_UNIT(*)
PLANE_ANGLE_UNIT()
SI_UNIT($,.RADIAN.)
);
#17117=(
NAMED_UNIT(*)
SI_UNIT($,.STERADIAN.)
SOLID_ANGLE_UNIT()
);
#17136=SHAPE_DEFINITION_REPRESENTATION(#17167,#17202);
#17167=PRODUCT_DEFINITION_SHAPE('',$,#17225);
#17202=SHAPE_REPRESENTATION('',(#6836,#253),#17109);
#17206=PRODUCT_DEFINITION_CONTEXT('part definition',#17274,'design');
#17225=PRODUCT_DEFINITION('6-1','6-1',#17247,#17206);
#17247=PRODUCT_DEFINITION_FORMATION('',$,#17294);
#17274=APPLICATION_CONTEXT(
'Core Data for Automotive Mechanical Design Process');
#17275=PRODUCT_CONTEXT('part definition',#17274,'mechanical');
#17294=PRODUCT('6-1','6-1','NOT SPECIFIED',(#17275));
#17298=PRESENTATION_STYLE_ASSIGNMENT((#17299));
#17299=SURFACE_STYLE_USAGE(.BOTH.,#17300);
#17300=SURFACE_SIDE_STYLE('',(#17301));
#17301=SURFACE_STYLE_FILL_AREA(#17302);
#17302=FILL_AREA_STYLE('Steel - Satin',(#17303));
#17303=FILL_AREA_STYLE_COLOUR('Steel - Satin',#17304);
#17304=COLOUR_RGB('Steel - Satin', 0.09019608, 0.27058824, 0.51372549);
ENDSEC;
END-ISO-10303-21;
